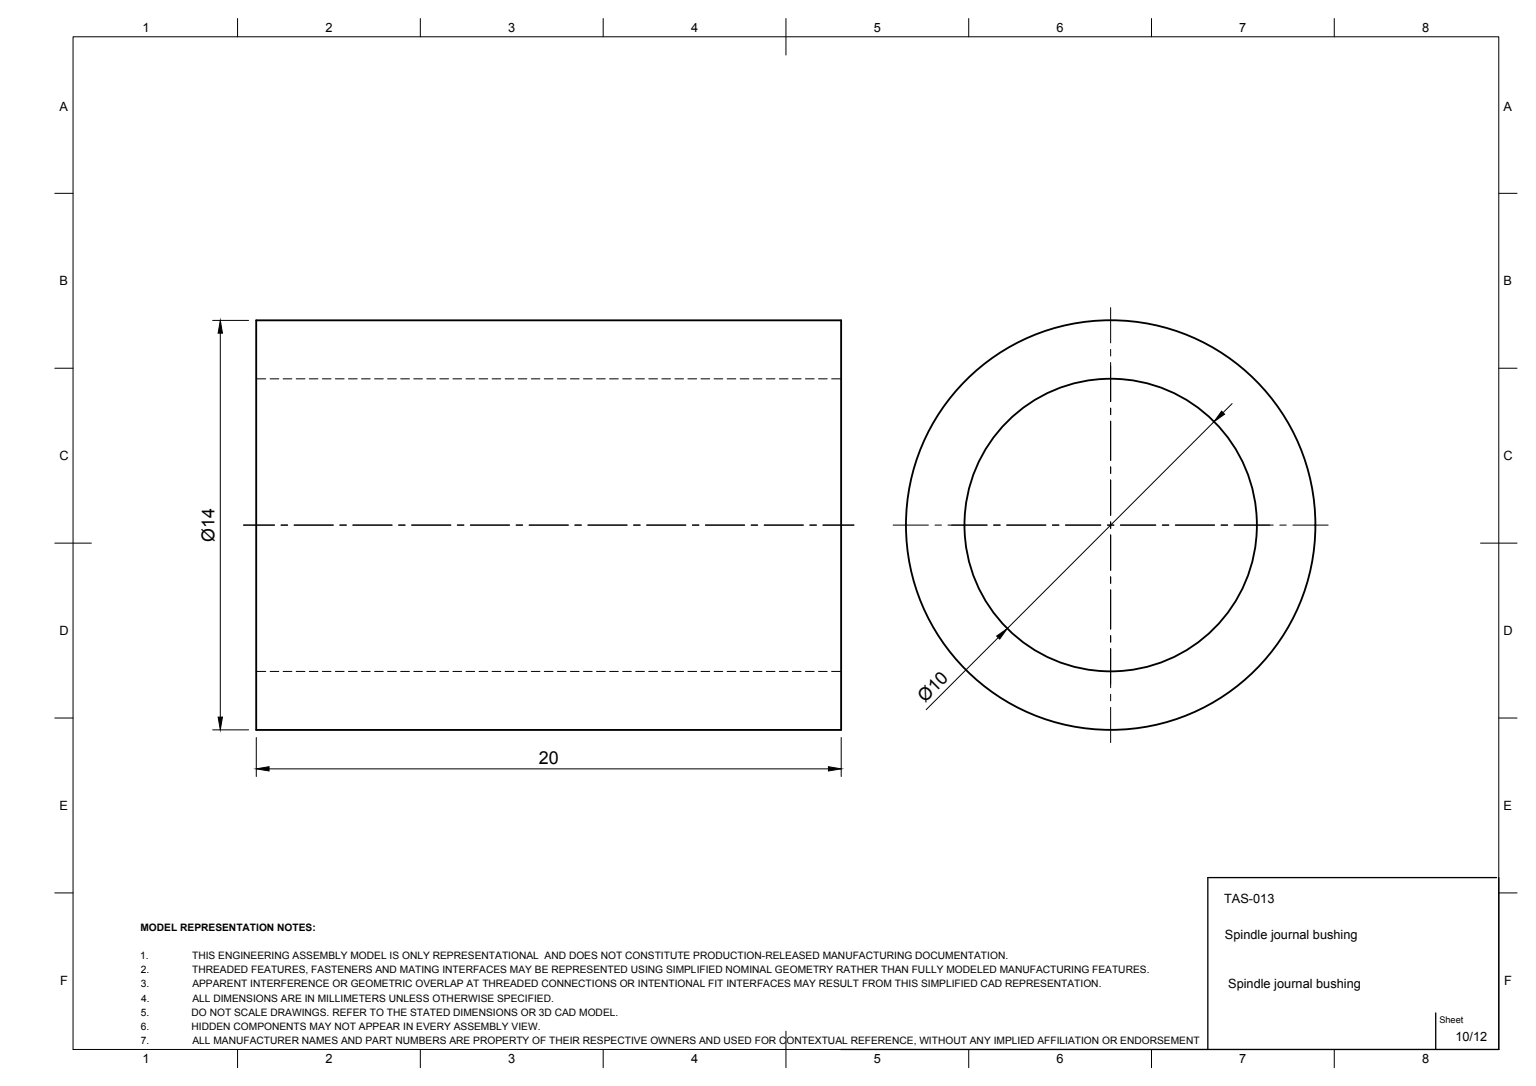
ISO-10303-21;
HEADER;
/* Generated by software containing ST-Developer
 * from STEP Tools, Inc. (www.steptools.com) 
 */

FILE_DESCRIPTION(
/* description */ (
'Independent guided parallel-jaw bracket clamp. Two12mm guide rods, re
placeable bronze sleeves, captured swiveling spindle, replaceable jaw 
pads and modeled M16x2 screw. Native slider/revolute joints linked2mm 
per revolution. Nominal opening0..122 with initial28mm. Base and two i
dentical supports welded. Standard fits, weld details and clamp load r
equire engineering selection.'),
/* implementation_level */ '2;1');

FILE_NAME(
/* name */ 'Spindle journal bushing.step',
/* time_stamp */ '2026-11-14T09:15:44-08:00',
/* author */ (''),
/* organization */ (''),
/* preprocessor_version */ 'ST-DEVELOPER v20.2',
/* originating_system */ 'Autodesk Translation Framework v15.17.0.0',
/* authorisation */ '');

FILE_SCHEMA (('AUTOMOTIVE_DESIGN { 1 0 10303 214 3 1 1 }'));
ENDSEC;

DATA;
#10=MECHANICAL_DESIGN_GEOMETRIC_PRESENTATION_REPRESENTATION('',(#917),#105806);
#893=SHAPE_REPRESENTATION_RELATIONSHIP('SRR','None',#105861,#905);
#905=ADVANCED_BREP_SHAPE_REPRESENTATION('',(#929),#105796);
#917=STYLED_ITEM('',(#105930),#929);
#929=MANIFOLD_SOLID_BREP('Body1',#7204);
#957=FACE_BOUND('',#1379,.T.);
#958=FACE_BOUND('',#1381,.T.);
#1010=PLANE('',#7396);
#1011=PLANE('',#7397);
#1086=FACE_OUTER_BOUND('',#1376,.T.);
#1087=FACE_OUTER_BOUND('',#1377,.T.);
#1088=FACE_OUTER_BOUND('',#1378,.T.);
#1089=FACE_OUTER_BOUND('',#1380,.T.);
#1376=EDGE_LOOP('',(#4515,#4516,#4517,#4518));
#1377=EDGE_LOOP('',(#4519,#4520,#4521,#4522));
#1378=EDGE_LOOP('',(#4523));
#1379=EDGE_LOOP('',(#4524));
#1380=EDGE_LOOP('',(#4525));
#1381=EDGE_LOOP('',(#4526));
#1701=LINE('',#8929,#1981);
#1702=LINE('',#8935,#1982);
#1981=VECTOR('',#7866,5.);
#1982=VECTOR('',#7873,7.);
#2246=CIRCLE('',#7391,5.);
#2247=CIRCLE('',#7392,5.);
#2248=CIRCLE('',#7394,7.);
#2249=CIRCLE('',#7395,7.);
#2360=VERTEX_POINT('',#8926);
#2361=VERTEX_POINT('',#8928);
#2362=VERTEX_POINT('',#8932);
#2363=VERTEX_POINT('',#8934);
#3302=EDGE_CURVE('',#2360,#2360,#2246,.T.);
#3303=EDGE_CURVE('',#2360,#2361,#1701,.T.);
#3304=EDGE_CURVE('',#2361,#2361,#2247,.T.);
#3305=EDGE_CURVE('',#2362,#2362,#2248,.T.);
#3306=EDGE_CURVE('',#2362,#2363,#1702,.T.);
#3307=EDGE_CURVE('',#2363,#2363,#2249,.T.);
#4515=ORIENTED_EDGE('',*,*,#3302,.T.);
#4516=ORIENTED_EDGE('',*,*,#3303,.T.);
#4517=ORIENTED_EDGE('',*,*,#3304,.F.);
#4518=ORIENTED_EDGE('',*,*,#3303,.F.);
#4519=ORIENTED_EDGE('',*,*,#3305,.F.);
#4520=ORIENTED_EDGE('',*,*,#3306,.T.);
#4521=ORIENTED_EDGE('',*,*,#3307,.T.);
#4522=ORIENTED_EDGE('',*,*,#3306,.F.);
#4523=ORIENTED_EDGE('',*,*,#3305,.T.);
#4524=ORIENTED_EDGE('',*,*,#3304,.T.);
#4525=ORIENTED_EDGE('',*,*,#3307,.F.);
#4526=ORIENTED_EDGE('',*,*,#3302,.F.);
#6746=CYLINDRICAL_SURFACE('',#7390,5.);
#6747=CYLINDRICAL_SURFACE('',#7393,7.);
#6951=ADVANCED_FACE('',(#1086),#6746,.F.);
#6952=ADVANCED_FACE('',(#1087),#6747,.T.);
#6953=ADVANCED_FACE('',(#1088,#957),#1010,.T.);
#6954=ADVANCED_FACE('',(#1089,#958),#1011,.F.);
#7204=CLOSED_SHELL('',(#6951,#6952,#6953,#6954));
#7389=AXIS2_PLACEMENT_3D('',#8924,#7860,#7861);
#7390=AXIS2_PLACEMENT_3D('',#8925,#7862,#7863);
#7391=AXIS2_PLACEMENT_3D('',#8927,#7864,#7865);
#7392=AXIS2_PLACEMENT_3D('',#8930,#7867,#7868);
#7393=AXIS2_PLACEMENT_3D('',#8931,#7869,#7870);
#7394=AXIS2_PLACEMENT_3D('',#8933,#7871,#7872);
#7395=AXIS2_PLACEMENT_3D('',#8936,#7874,#7875);
#7396=AXIS2_PLACEMENT_3D('',#8937,#7876,#7877);
#7397=AXIS2_PLACEMENT_3D('',#8938,#7878,#7879);
#7860=DIRECTION('axis',(0.,0.,1.));
#7861=DIRECTION('refdir',(1.,0.,0.));
#7862=DIRECTION('center_axis',(0.,0.,1.));
#7863=DIRECTION('ref_axis',(1.,0.,0.));
#7864=DIRECTION('center_axis',(0.,0.,-1.));
#7865=DIRECTION('ref_axis',(1.,0.,0.));
#7866=DIRECTION('',(0.,0.,1.));
#7867=DIRECTION('center_axis',(0.,0.,-1.));
#7868=DIRECTION('ref_axis',(1.,0.,0.));
#7869=DIRECTION('center_axis',(0.,0.,1.));
#7870=DIRECTION('ref_axis',(1.,0.,0.));
#7871=DIRECTION('center_axis',(0.,0.,1.));
#7872=DIRECTION('ref_axis',(1.,0.,0.));
#7873=DIRECTION('',(0.,0.,-1.));
#7874=DIRECTION('center_axis',(0.,0.,1.));
#7875=DIRECTION('ref_axis',(1.,0.,0.));
#7876=DIRECTION('center_axis',(0.,0.,1.));
#7877=DIRECTION('ref_axis',(1.,0.,0.));
#7878=DIRECTION('center_axis',(0.,0.,1.));
#7879=DIRECTION('ref_axis',(1.,0.,0.));
#8924=CARTESIAN_POINT('',(0.,0.,0.));
#8925=CARTESIAN_POINT('Origin',(0.,0.,0.));
#8926=CARTESIAN_POINT('',(-5.,-6.12323399573677E-16,0.));
#8927=CARTESIAN_POINT('Origin',(0.,0.,0.));
#8928=CARTESIAN_POINT('',(-5.,-6.12323399573677E-16,20.));
#8929=CARTESIAN_POINT('',(-5.,-6.12323399573677E-16,0.));
#8930=CARTESIAN_POINT('Origin',(0.,0.,20.));
#8931=CARTESIAN_POINT('Origin',(0.,0.,0.));
#8932=CARTESIAN_POINT('',(-7.,-8.57252759403147E-16,20.));
#8933=CARTESIAN_POINT('Origin',(0.,0.,20.));
#8934=CARTESIAN_POINT('',(-7.,-8.57252759403147E-16,0.));
#8935=CARTESIAN_POINT('',(-7.,-8.57252759403147E-16,0.));
#8936=CARTESIAN_POINT('Origin',(0.,0.,0.));
#8937=CARTESIAN_POINT('Origin',(0.,0.,20.));
#8938=CARTESIAN_POINT('Origin',(0.,0.,0.));
#105782=UNCERTAINTY_MEASURE_WITH_UNIT(LENGTH_MEASURE(0.01),#105807,
'DISTANCE_ACCURACY_VALUE',
'Maximum model space distance between geometric entities at asserted c
onnectivities');
#105792=UNCERTAINTY_MEASURE_WITH_UNIT(LENGTH_MEASURE(0.01),#105807,
'DISTANCE_ACCURACY_VALUE',
'Maximum model space distance between geometric entities at asserted c
onnectivities');
#105796=(
GEOMETRIC_REPRESENTATION_CONTEXT(3)
GLOBAL_UNCERTAINTY_ASSIGNED_CONTEXT((#105782))
GLOBAL_UNIT_ASSIGNED_CONTEXT((#105807,#105809,#105810))
REPRESENTATION_CONTEXT('','3D')
);
#105806=(
GEOMETRIC_REPRESENTATION_CONTEXT(3)
GLOBAL_UNCERTAINTY_ASSIGNED_CONTEXT((#105792))
GLOBAL_UNIT_ASSIGNED_CONTEXT((#105807,#105809,#105810))
REPRESENTATION_CONTEXT('','3D')
);
#105807=(
LENGTH_UNIT()
NAMED_UNIT(*)
SI_UNIT(.MILLI.,.METRE.)
);
#105809=(
NAMED_UNIT(*)
PLANE_ANGLE_UNIT()
SI_UNIT($,.RADIAN.)
);
#105810=(
NAMED_UNIT(*)
SI_UNIT($,.STERADIAN.)
SOLID_ANGLE_UNIT()
);
#105814=SHAPE_DEFINITION_REPRESENTATION(#105827,#105861);
#105827=PRODUCT_DEFINITION_SHAPE('',$,#105875);
#105861=SHAPE_REPRESENTATION('',(#7389),#105796);
#105871=PRODUCT_DEFINITION_CONTEXT('part definition',#105912,'design');
#105875=PRODUCT_DEFINITION('Spindle journal bushing',
'Spindle journal bushing',#105888,#105871);
#105888=PRODUCT_DEFINITION_FORMATION('',$,#105917);
#105912=APPLICATION_CONTEXT(
'Core Data for Automotive Mechanical Design Process');
#105913=PRODUCT_CONTEXT('part definition',#105912,'mechanical');
#105917=PRODUCT('Spindle journal bushing','Spindle journal bushing',$,(#105913));
#105930=PRESENTATION_STYLE_ASSIGNMENT((#105936));
#105936=SURFACE_STYLE_USAGE(.BOTH.,#105942);
#105942=SURFACE_SIDE_STYLE('',(#105948));
#105948=SURFACE_STYLE_FILL_AREA(#105954);
#105954=FILL_AREA_STYLE('Opaque(185,192,202)',(#105960));
#105960=FILL_AREA_STYLE_COLOUR('Opaque(185,192,202)',#105966);
#105966=COLOUR_RGB('Opaque(185,192,202)',0.725490196078431,0.752941176470588,
0.792156862745098);
ENDSEC;
END-ISO-10303-21;
